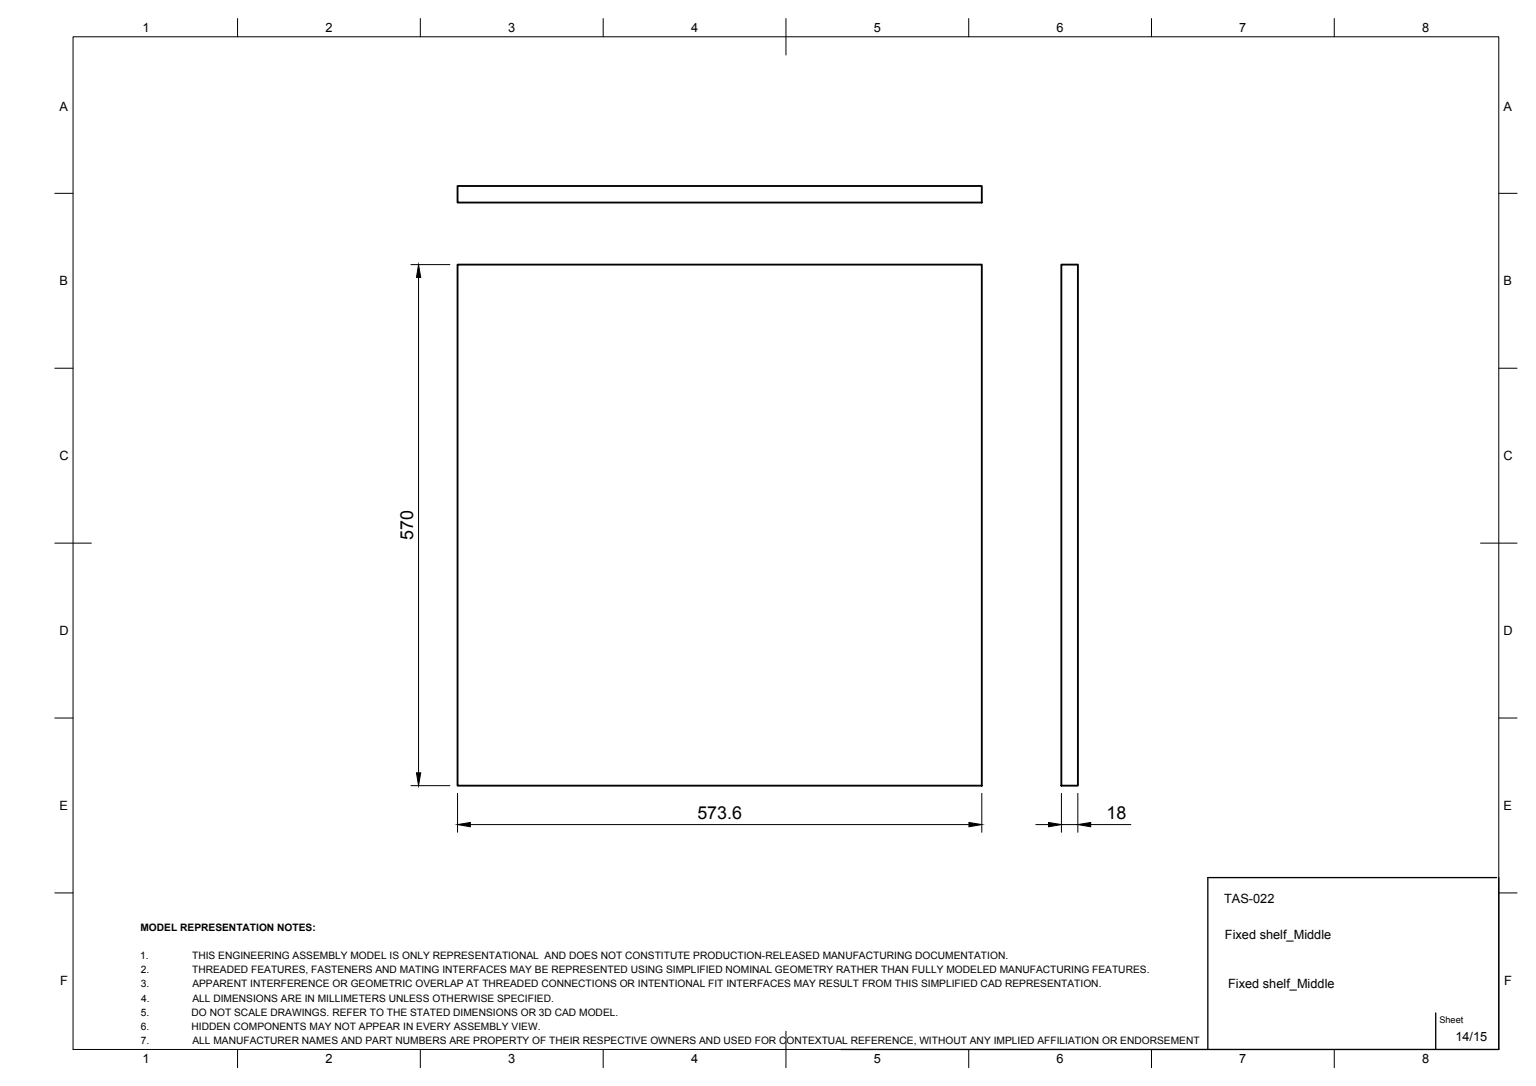
ISO-10303-21;
HEADER;
/* Generated by software containing ST-Developer
 * from STEP Tools, Inc. (www.steptools.com) 
 */

FILE_DESCRIPTION(
/* description */ (''),
/* implementation_level */ '2;1');

FILE_NAME(
/* name */ 'Fixed shelf_Middle.step',
/* time_stamp */ '2026-11-15T21:02:08-08:00',
/* author */ (''),
/* organization */ (''),
/* preprocessor_version */ 'ST-DEVELOPER v20.2',
/* originating_system */ 'Autodesk Translation Framework v15.17.0.0',
/* authorisation */ '');

FILE_SCHEMA (('AUTOMOTIVE_DESIGN { 1 0 10303 214 3 1 1 }'));
ENDSEC;

DATA;
#10=MECHANICAL_DESIGN_GEOMETRIC_PRESENTATION_REPRESENTATION('',(#615),#31566);
#585=SHAPE_REPRESENTATION_RELATIONSHIP('SRR','None',#31649,#600);
#600=ADVANCED_BREP_SHAPE_REPRESENTATION('',(#630),#31564);
#615=STYLED_ITEM('',(#31721),#630);
#630=MANIFOLD_SOLID_BREP('Body1',#5728);
#892=FACE_OUTER_BOUND('',#1197,.T.);
#893=FACE_OUTER_BOUND('',#1198,.T.);
#894=FACE_OUTER_BOUND('',#1199,.T.);
#895=FACE_OUTER_BOUND('',#1200,.T.);
#896=FACE_OUTER_BOUND('',#1201,.T.);
#897=FACE_OUTER_BOUND('',#1202,.T.);
#1197=EDGE_LOOP('',(#5233,#5234,#5235,#5236));
#1198=EDGE_LOOP('',(#5237,#5238,#5239,#5240));
#1199=EDGE_LOOP('',(#5241,#5242,#5243,#5244));
#1200=EDGE_LOOP('',(#5245,#5246,#5247,#5248));
#1201=EDGE_LOOP('',(#5249,#5250,#5251,#5252));
#1202=EDGE_LOOP('',(#5253,#5254,#5255,#5256));
#1700=LINE('',#31469,#2207);
#1701=LINE('',#31471,#2208);
#1702=LINE('',#31473,#2209);
#1703=LINE('',#31474,#2210);
#1704=LINE('',#31477,#2211);
#1705=LINE('',#31479,#2212);
#1706=LINE('',#31480,#2213);
#1707=LINE('',#31483,#2214);
#1708=LINE('',#31485,#2215);
#1709=LINE('',#31486,#2216);
#1710=LINE('',#31488,#2217);
#1711=LINE('',#31489,#2218);
#2207=VECTOR('',#7462,1.);
#2208=VECTOR('',#7463,1.);
#2209=VECTOR('',#7464,1.);
#2210=VECTOR('',#7465,1.);
#2211=VECTOR('',#7468,1.);
#2212=VECTOR('',#7469,1.);
#2213=VECTOR('',#7470,1.);
#2214=VECTOR('',#7473,1.);
#2215=VECTOR('',#7474,1.);
#2216=VECTOR('',#7475,1.);
#2217=VECTOR('',#7478,1.);
#2218=VECTOR('',#7479,1.);
#2799=VERTEX_POINT('',#31467);
#2800=VERTEX_POINT('',#31468);
#2801=VERTEX_POINT('',#31470);
#2802=VERTEX_POINT('',#31472);
#2803=VERTEX_POINT('',#31476);
#2804=VERTEX_POINT('',#31478);
#2805=VERTEX_POINT('',#31482);
#2806=VERTEX_POINT('',#31484);
#3612=EDGE_CURVE('',#2799,#2800,#1700,.T.);
#3613=EDGE_CURVE('',#2800,#2801,#1701,.T.);
#3614=EDGE_CURVE('',#2802,#2801,#1702,.T.);
#3615=EDGE_CURVE('',#2799,#2802,#1703,.T.);
#3616=EDGE_CURVE('',#2803,#2799,#1704,.T.);
#3617=EDGE_CURVE('',#2804,#2802,#1705,.T.);
#3618=EDGE_CURVE('',#2803,#2804,#1706,.T.);
#3619=EDGE_CURVE('',#2805,#2803,#1707,.T.);
#3620=EDGE_CURVE('',#2806,#2804,#1708,.T.);
#3621=EDGE_CURVE('',#2805,#2806,#1709,.T.);
#3622=EDGE_CURVE('',#2800,#2805,#1710,.T.);
#3623=EDGE_CURVE('',#2801,#2806,#1711,.T.);
#5233=ORIENTED_EDGE('',*,*,#3612,.T.);
#5234=ORIENTED_EDGE('',*,*,#3613,.T.);
#5235=ORIENTED_EDGE('',*,*,#3614,.F.);
#5236=ORIENTED_EDGE('',*,*,#3615,.F.);
#5237=ORIENTED_EDGE('',*,*,#3616,.T.);
#5238=ORIENTED_EDGE('',*,*,#3615,.T.);
#5239=ORIENTED_EDGE('',*,*,#3617,.F.);
#5240=ORIENTED_EDGE('',*,*,#3618,.F.);
#5241=ORIENTED_EDGE('',*,*,#3619,.T.);
#5242=ORIENTED_EDGE('',*,*,#3618,.T.);
#5243=ORIENTED_EDGE('',*,*,#3620,.F.);
#5244=ORIENTED_EDGE('',*,*,#3621,.F.);
#5245=ORIENTED_EDGE('',*,*,#3622,.T.);
#5246=ORIENTED_EDGE('',*,*,#3621,.T.);
#5247=ORIENTED_EDGE('',*,*,#3623,.F.);
#5248=ORIENTED_EDGE('',*,*,#3613,.F.);
#5249=ORIENTED_EDGE('',*,*,#3623,.T.);
#5250=ORIENTED_EDGE('',*,*,#3620,.T.);
#5251=ORIENTED_EDGE('',*,*,#3617,.T.);
#5252=ORIENTED_EDGE('',*,*,#3614,.T.);
#5253=ORIENTED_EDGE('',*,*,#3622,.F.);
#5254=ORIENTED_EDGE('',*,*,#3612,.F.);
#5255=ORIENTED_EDGE('',*,*,#3616,.F.);
#5256=ORIENTED_EDGE('',*,*,#3619,.F.);
#5438=PLANE('',#6238);
#5439=PLANE('',#6239);
#5440=PLANE('',#6240);
#5441=PLANE('',#6241);
#5442=PLANE('',#6242);
#5443=PLANE('',#6243);
#5706=ADVANCED_FACE('',(#892),#5438,.T.);
#5707=ADVANCED_FACE('',(#893),#5439,.T.);
#5708=ADVANCED_FACE('',(#894),#5440,.T.);
#5709=ADVANCED_FACE('',(#895),#5441,.T.);
#5710=ADVANCED_FACE('',(#896),#5442,.T.);
#5711=ADVANCED_FACE('',(#897),#5443,.F.);
#5728=CLOSED_SHELL('',(#5706,#5707,#5708,#5709,#5710,#5711));
#6237=AXIS2_PLACEMENT_3D('',#31465,#7458,#7459);
#6238=AXIS2_PLACEMENT_3D('',#31466,#7460,#7461);
#6239=AXIS2_PLACEMENT_3D('',#31475,#7466,#7467);
#6240=AXIS2_PLACEMENT_3D('',#31481,#7471,#7472);
#6241=AXIS2_PLACEMENT_3D('',#31487,#7476,#7477);
#6242=AXIS2_PLACEMENT_3D('',#31490,#7480,#7481);
#6243=AXIS2_PLACEMENT_3D('',#31491,#7482,#7483);
#7458=DIRECTION('axis',(0.,0.,1.));
#7459=DIRECTION('refdir',(1.,0.,0.));
#7460=DIRECTION('center_axis',(0.,1.,0.));
#7461=DIRECTION('ref_axis',(-1.,0.,0.));
#7462=DIRECTION('',(-1.,0.,0.));
#7463=DIRECTION('',(0.,0.,1.));
#7464=DIRECTION('',(-1.,0.,0.));
#7465=DIRECTION('',(0.,0.,1.));
#7466=DIRECTION('center_axis',(1.,0.,0.));
#7467=DIRECTION('ref_axis',(0.,1.,0.));
#7468=DIRECTION('',(0.,1.,0.));
#7469=DIRECTION('',(0.,1.,0.));
#7470=DIRECTION('',(0.,0.,1.));
#7471=DIRECTION('center_axis',(0.,-1.,0.));
#7472=DIRECTION('ref_axis',(1.,0.,0.));
#7473=DIRECTION('',(1.,0.,0.));
#7474=DIRECTION('',(1.,0.,0.));
#7475=DIRECTION('',(0.,0.,1.));
#7476=DIRECTION('center_axis',(-1.,0.,0.));
#7477=DIRECTION('ref_axis',(0.,-1.,0.));
#7478=DIRECTION('',(0.,-1.,0.));
#7479=DIRECTION('',(0.,-1.,0.));
#7480=DIRECTION('center_axis',(0.,0.,1.));
#7481=DIRECTION('ref_axis',(1.,0.,0.));
#7482=DIRECTION('center_axis',(0.,0.,1.));
#7483=DIRECTION('ref_axis',(1.,0.,0.));
#31465=CARTESIAN_POINT('',(0.,0.,0.));
#31466=CARTESIAN_POINT('Origin',(57.36,57.6,0.));
#31467=CARTESIAN_POINT('',(57.36,57.6,0.));
#31468=CARTESIAN_POINT('',(0.,57.6,0.));
#31469=CARTESIAN_POINT('',(57.36,57.6,0.));
#31470=CARTESIAN_POINT('',(0.,57.6,1.8));
#31471=CARTESIAN_POINT('',(0.,57.6,0.));
#31472=CARTESIAN_POINT('',(57.36,57.6,1.8));
#31473=CARTESIAN_POINT('',(57.36,57.6,1.8));
#31474=CARTESIAN_POINT('',(57.36,57.6,0.));
#31475=CARTESIAN_POINT('Origin',(57.36,0.6,0.));
#31476=CARTESIAN_POINT('',(57.36,0.6,0.));
#31477=CARTESIAN_POINT('',(57.36,0.6,0.));
#31478=CARTESIAN_POINT('',(57.36,0.600000000000001,1.8));
#31479=CARTESIAN_POINT('',(57.36,0.6,1.8));
#31480=CARTESIAN_POINT('',(57.36,0.6,0.));
#31481=CARTESIAN_POINT('Origin',(0.,0.6,0.));
#31482=CARTESIAN_POINT('',(0.,0.600000000000001,0.));
#31483=CARTESIAN_POINT('',(0.,0.6,0.));
#31484=CARTESIAN_POINT('',(0.,0.600000000000001,1.8));
#31485=CARTESIAN_POINT('',(0.,0.6,1.8));
#31486=CARTESIAN_POINT('',(0.,0.600000000000001,0.));
#31487=CARTESIAN_POINT('Origin',(0.,57.6,0.));
#31488=CARTESIAN_POINT('',(0.,57.6,0.));
#31489=CARTESIAN_POINT('',(0.,57.6,1.8));
#31490=CARTESIAN_POINT('Origin',(28.68,29.1,1.8));
#31491=CARTESIAN_POINT('Origin',(28.68,29.1,0.));
#31547=UNCERTAINTY_MEASURE_WITH_UNIT(LENGTH_MEASURE(0.001),#31567,
'DISTANCE_ACCURACY_VALUE',
'Maximum model space distance between geometric entities at asserted c
onnectivities');
#31549=UNCERTAINTY_MEASURE_WITH_UNIT(LENGTH_MEASURE(0.001),#31567,
'DISTANCE_ACCURACY_VALUE',
'Maximum model space distance between geometric entities at asserted c
onnectivities');
#31564=(
GEOMETRIC_REPRESENTATION_CONTEXT(3)
GLOBAL_UNCERTAINTY_ASSIGNED_CONTEXT((#31547))
GLOBAL_UNIT_ASSIGNED_CONTEXT((#31567,#31569,#31570))
REPRESENTATION_CONTEXT('','3D')
);
#31566=(
GEOMETRIC_REPRESENTATION_CONTEXT(3)
GLOBAL_UNCERTAINTY_ASSIGNED_CONTEXT((#31549))
GLOBAL_UNIT_ASSIGNED_CONTEXT((#31567,#31569,#31570))
REPRESENTATION_CONTEXT('','3D')
);
#31567=(
LENGTH_UNIT()
NAMED_UNIT(*)
SI_UNIT(.CENTI.,.METRE.)
);
#31569=(
NAMED_UNIT(*)
PLANE_ANGLE_UNIT()
SI_UNIT($,.RADIAN.)
);
#31570=(
NAMED_UNIT(*)
SI_UNIT($,.STERADIAN.)
SOLID_ANGLE_UNIT()
);
#31585=SHAPE_DEFINITION_REPRESENTATION(#31601,#31649);
#31601=PRODUCT_DEFINITION_SHAPE('',$,#31666);
#31649=SHAPE_REPRESENTATION('',(#6237),#31564);
#31651=PRODUCT_DEFINITION_CONTEXT('part definition',#31701,'design');
#31666=PRODUCT_DEFINITION('Fixed shelf_Middle','Fixed shelf_Middle',#31682,
#31651);
#31682=PRODUCT_DEFINITION_FORMATION('',$,#31717);
#31701=APPLICATION_CONTEXT(
'Core Data for Automotive Mechanical Design Process');
#31702=PRODUCT_CONTEXT('part definition',#31701,'mechanical');
#31717=PRODUCT('Fixed shelf_Middle','Fixed shelf_Middle',$,(#31702));
#31721=PRESENTATION_STYLE_ASSIGNMENT((#31728));
#31728=SURFACE_STYLE_USAGE(.BOTH.,#31735);
#31735=SURFACE_SIDE_STYLE('',(#31742));
#31742=SURFACE_STYLE_FILL_AREA(#31749);
#31749=FILL_AREA_STYLE('Opaque(70,153,204)',(#31756));
#31756=FILL_AREA_STYLE_COLOUR('Opaque(70,153,204)',#31763);
#31763=COLOUR_RGB('Opaque(70,153,204)',0.274509803921569,0.6,0.8);
ENDSEC;
END-ISO-10303-21;
